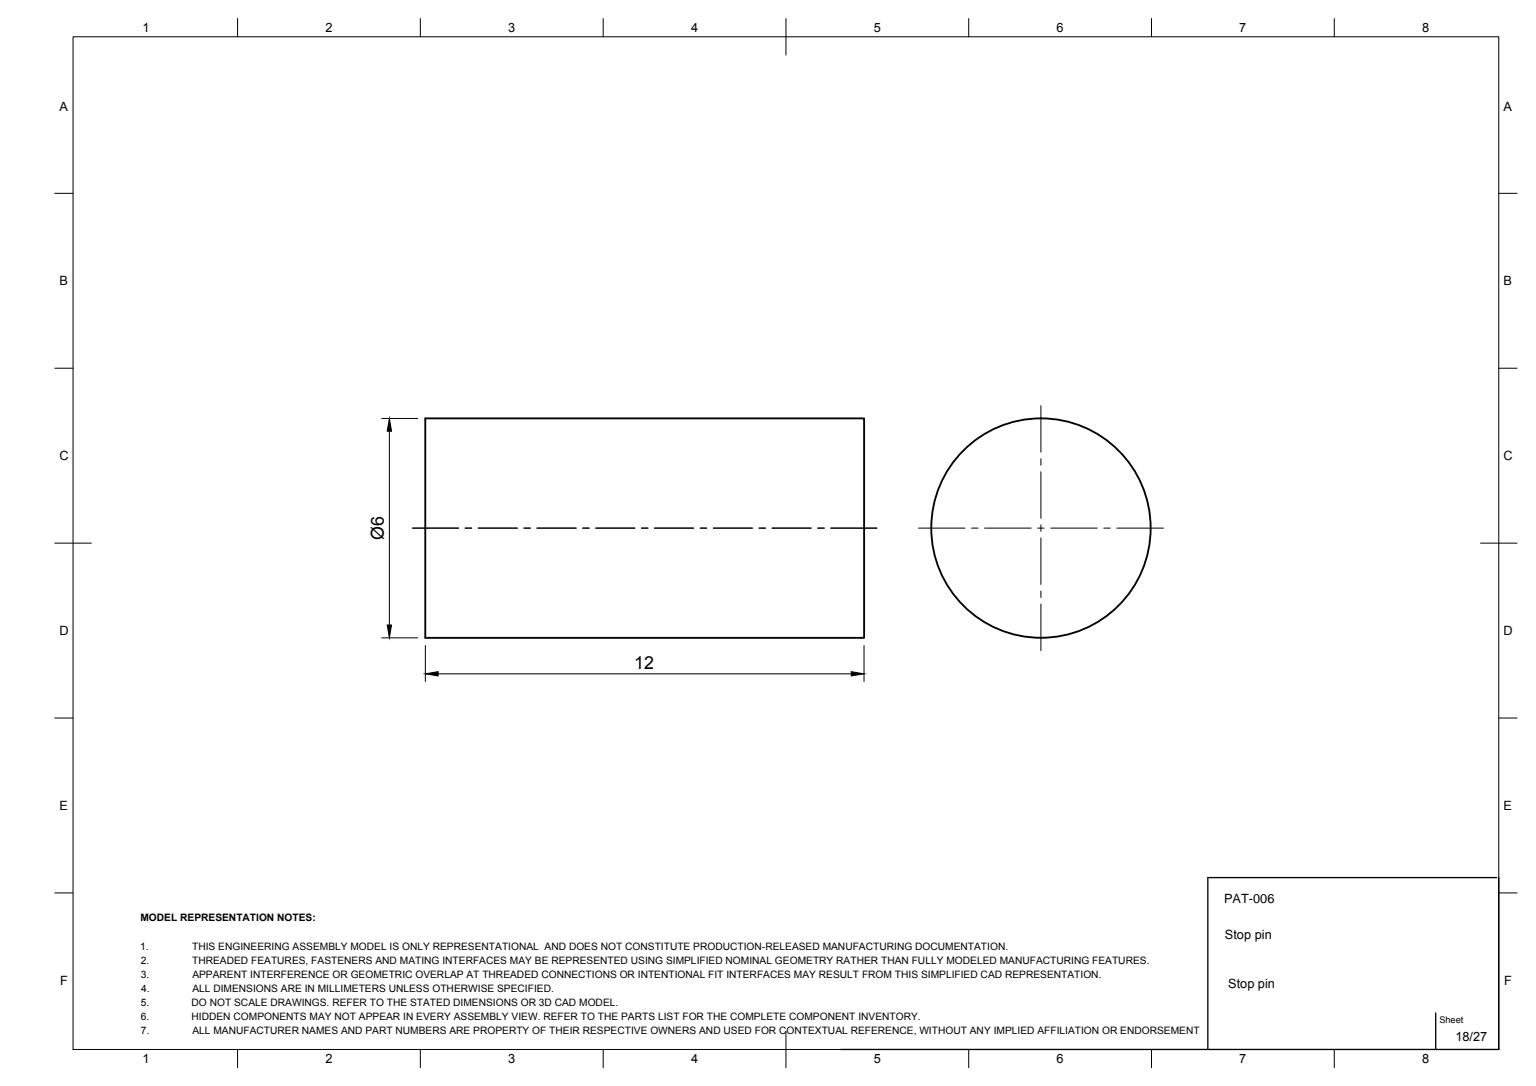
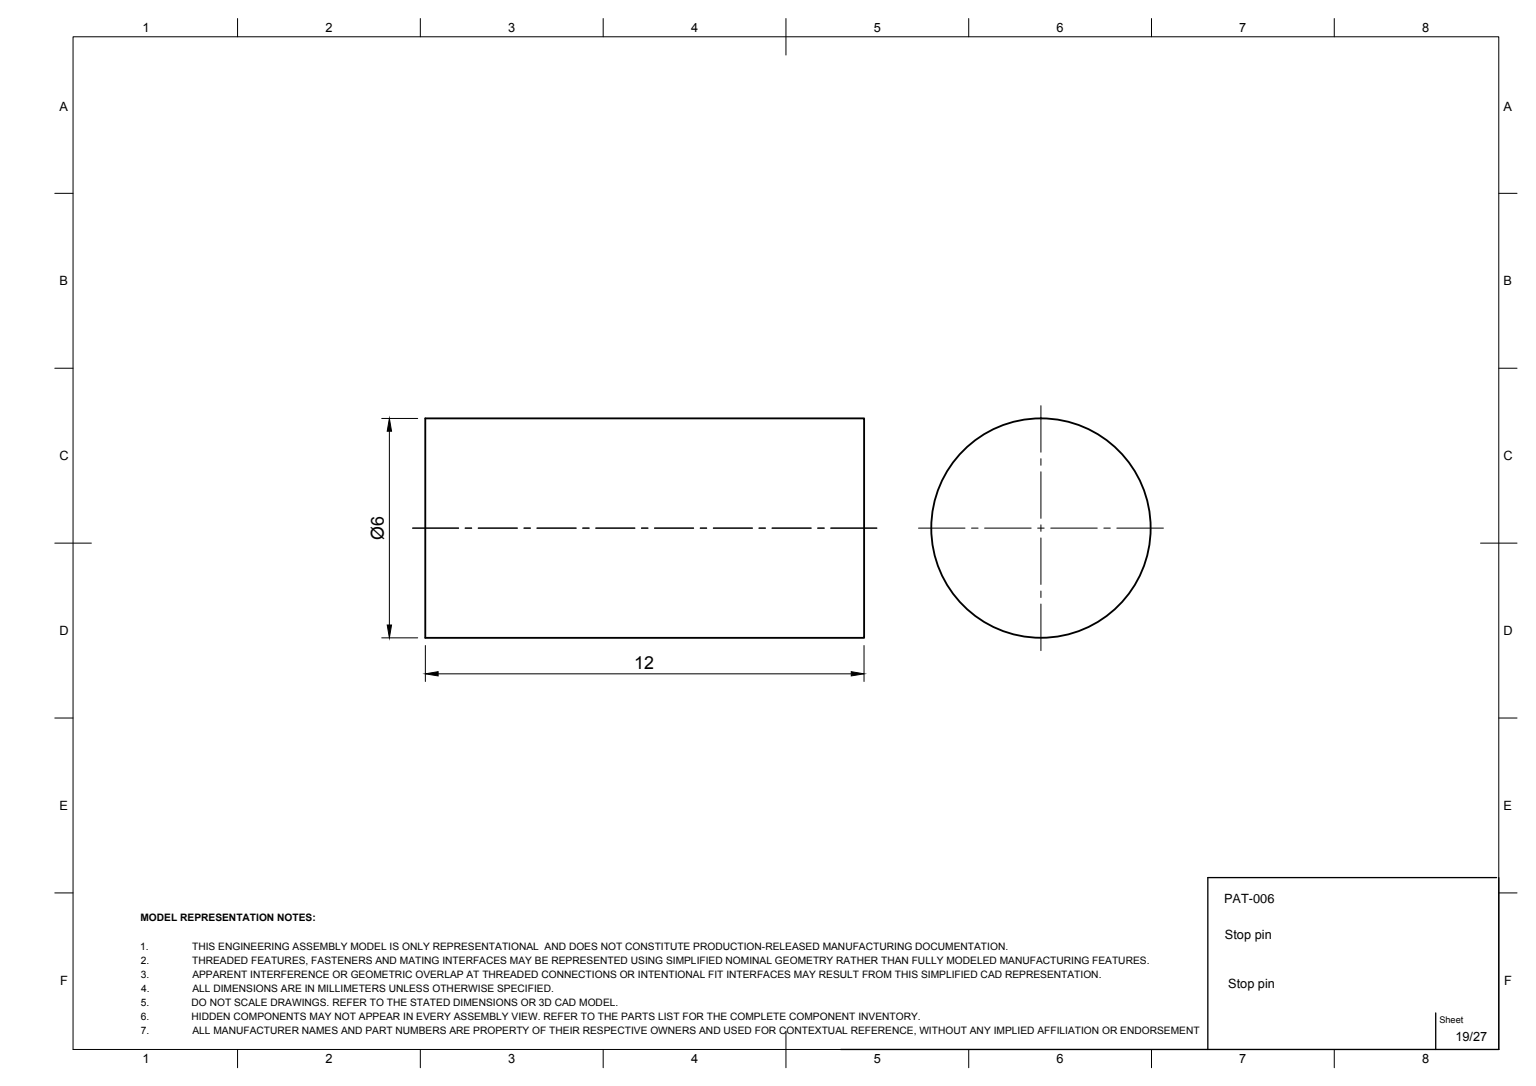
ISO-10303-21;
HEADER;
/* Generated by software containing ST-Developer
 * from STEP Tools, Inc. (www.steptools.com) 
 */

FILE_DESCRIPTION(
/* description */ ('Ball-type isolation valve (generic)'),
/* implementation_level */ '2;1');

FILE_NAME(
/* name */ 'Stop pin.step',
/* time_stamp */ '2026-10-27T10:53:05-07:00',
/* author */ (''),
/* organization */ (''),
/* preprocessor_version */ 'ST-DEVELOPER v20.2',
/* originating_system */ 'Autodesk Translation Framework v15.17.0.0',
/* authorisation */ '');

FILE_SCHEMA (('AUTOMOTIVE_DESIGN { 1 0 10303 214 3 1 1 }'));
ENDSEC;

DATA;
#10=MECHANICAL_DESIGN_GEOMETRIC_PRESENTATION_REPRESENTATION('',(#290),#7425);
#238=SHAPE_REPRESENTATION_RELATIONSHIP('SRR','None',#7548,#264);
#264=ADVANCED_BREP_SHAPE_REPRESENTATION('',(#316),#7411);
#290=STYLED_ITEM('',(#7744),#316);
#316=MANIFOLD_SOLID_BREP('Body1',#4095);
#478=PLANE('',#4635);
#479=PLANE('',#4636);
#691=FACE_OUTER_BOUND('',#1008,.T.);
#692=FACE_OUTER_BOUND('',#1009,.T.);
#693=FACE_OUTER_BOUND('',#1010,.T.);
#1008=EDGE_LOOP('',(#3225,#3226,#3227,#3228));
#1009=EDGE_LOOP('',(#3229));
#1010=EDGE_LOOP('',(#3230));
#1284=LINE('',#6708,#1592);
#1592=VECTOR('',#5487,0.3);
#1887=CIRCLE('',#4633,0.3);
#1888=CIRCLE('',#4634,0.3);
#2107=VERTEX_POINT('',#6705);
#2108=VERTEX_POINT('',#6707);
#2505=EDGE_CURVE('',#2107,#2107,#1887,.T.);
#2506=EDGE_CURVE('',#2107,#2108,#1284,.T.);
#2507=EDGE_CURVE('',#2108,#2108,#1888,.T.);
#3225=ORIENTED_EDGE('',*,*,#2505,.F.);
#3226=ORIENTED_EDGE('',*,*,#2506,.T.);
#3227=ORIENTED_EDGE('',*,*,#2507,.T.);
#3228=ORIENTED_EDGE('',*,*,#2506,.F.);
#3229=ORIENTED_EDGE('',*,*,#2505,.T.);
#3230=ORIENTED_EDGE('',*,*,#2507,.F.);
#3813=CYLINDRICAL_SURFACE('',#4632,0.3);
#3945=ADVANCED_FACE('',(#691),#3813,.T.);
#3946=ADVANCED_FACE('',(#692),#478,.T.);
#3947=ADVANCED_FACE('',(#693),#479,.F.);
#4095=CLOSED_SHELL('',(#3945,#3946,#3947));
#4631=AXIS2_PLACEMENT_3D('',#6703,#5481,#5482);
#4632=AXIS2_PLACEMENT_3D('',#6704,#5483,#5484);
#4633=AXIS2_PLACEMENT_3D('',#6706,#5485,#5486);
#4634=AXIS2_PLACEMENT_3D('',#6709,#5488,#5489);
#4635=AXIS2_PLACEMENT_3D('',#6710,#5490,#5491);
#4636=AXIS2_PLACEMENT_3D('',#6711,#5492,#5493);
#5481=DIRECTION('axis',(0.,0.,1.));
#5482=DIRECTION('refdir',(1.,0.,0.));
#5483=DIRECTION('center_axis',(0.,0.,1.));
#5484=DIRECTION('ref_axis',(1.,0.,0.));
#5485=DIRECTION('center_axis',(0.,0.,1.));
#5486=DIRECTION('ref_axis',(1.,0.,0.));
#5487=DIRECTION('',(0.,0.,-1.));
#5488=DIRECTION('center_axis',(0.,0.,1.));
#5489=DIRECTION('ref_axis',(1.,0.,0.));
#5490=DIRECTION('center_axis',(0.,0.,1.));
#5491=DIRECTION('ref_axis',(1.,0.,0.));
#5492=DIRECTION('center_axis',(0.,0.,1.));
#5493=DIRECTION('ref_axis',(1.,0.,0.));
#6703=CARTESIAN_POINT('',(0.,0.,0.));
#6704=CARTESIAN_POINT('Origin',(3.,1.1,8.2));
#6705=CARTESIAN_POINT('',(2.7,1.1,9.4));
#6706=CARTESIAN_POINT('Origin',(3.,1.1,9.4));
#6707=CARTESIAN_POINT('',(2.7,1.1,8.2));
#6708=CARTESIAN_POINT('',(2.7,1.1,8.2));
#6709=CARTESIAN_POINT('Origin',(3.,1.1,8.2));
#6710=CARTESIAN_POINT('Origin',(3.,1.1,9.4));
#6711=CARTESIAN_POINT('Origin',(3.,1.1,8.2));
#7381=UNCERTAINTY_MEASURE_WITH_UNIT(LENGTH_MEASURE(0.001),#7426,
'DISTANCE_ACCURACY_VALUE',
'Maximum model space distance between geometric entities at asserted c
onnectivities');
#7395=UNCERTAINTY_MEASURE_WITH_UNIT(LENGTH_MEASURE(0.001),#7426,
'DISTANCE_ACCURACY_VALUE',
'Maximum model space distance between geometric entities at asserted c
onnectivities');
#7411=(
GEOMETRIC_REPRESENTATION_CONTEXT(3)
GLOBAL_UNCERTAINTY_ASSIGNED_CONTEXT((#7381))
GLOBAL_UNIT_ASSIGNED_CONTEXT((#7426,#7428,#7429))
REPRESENTATION_CONTEXT('','3D')
);
#7425=(
GEOMETRIC_REPRESENTATION_CONTEXT(3)
GLOBAL_UNCERTAINTY_ASSIGNED_CONTEXT((#7395))
GLOBAL_UNIT_ASSIGNED_CONTEXT((#7426,#7428,#7429))
REPRESENTATION_CONTEXT('','3D')
);
#7426=(
LENGTH_UNIT()
NAMED_UNIT(*)
SI_UNIT(.CENTI.,.METRE.)
);
#7428=(
NAMED_UNIT(*)
PLANE_ANGLE_UNIT()
SI_UNIT($,.RADIAN.)
);
#7429=(
NAMED_UNIT(*)
SI_UNIT($,.STERADIAN.)
SOLID_ANGLE_UNIT()
);
#7445=SHAPE_DEFINITION_REPRESENTATION(#7474,#7548);
#7474=PRODUCT_DEFINITION_SHAPE('',$,#7578);
#7548=SHAPE_REPRESENTATION('',(#4631),#7411);
#7562=PRODUCT_DEFINITION_CONTEXT('part definition',#7651,'design');
#7578=PRODUCT_DEFINITION('Stop pin','Stop pin',#7607,#7562);
#7607=PRODUCT_DEFINITION_FORMATION('',$,#7668);
#7651=APPLICATION_CONTEXT(
'Core Data for Automotive Mechanical Design Process');
#7652=PRODUCT_CONTEXT('part definition',#7651,'mechanical');
#7668=PRODUCT('Stop pin','Stop pin','Stop pin',(#7652));
#7738=COLOUR_RGB('Grey',0.48,0.52,0.57);
#7739=FILL_AREA_STYLE_COLOUR('',#7738);
#7740=FILL_AREA_STYLE('',(#7739));
#7741=SURFACE_STYLE_FILL_AREA(#7740);
#7742=SURFACE_SIDE_STYLE('',(#7741));
#7743=SURFACE_STYLE_USAGE(.BOTH.,#7742);
#7744=PRESENTATION_STYLE_ASSIGNMENT((#7743));
ENDSEC;
END-ISO-10303-21;
